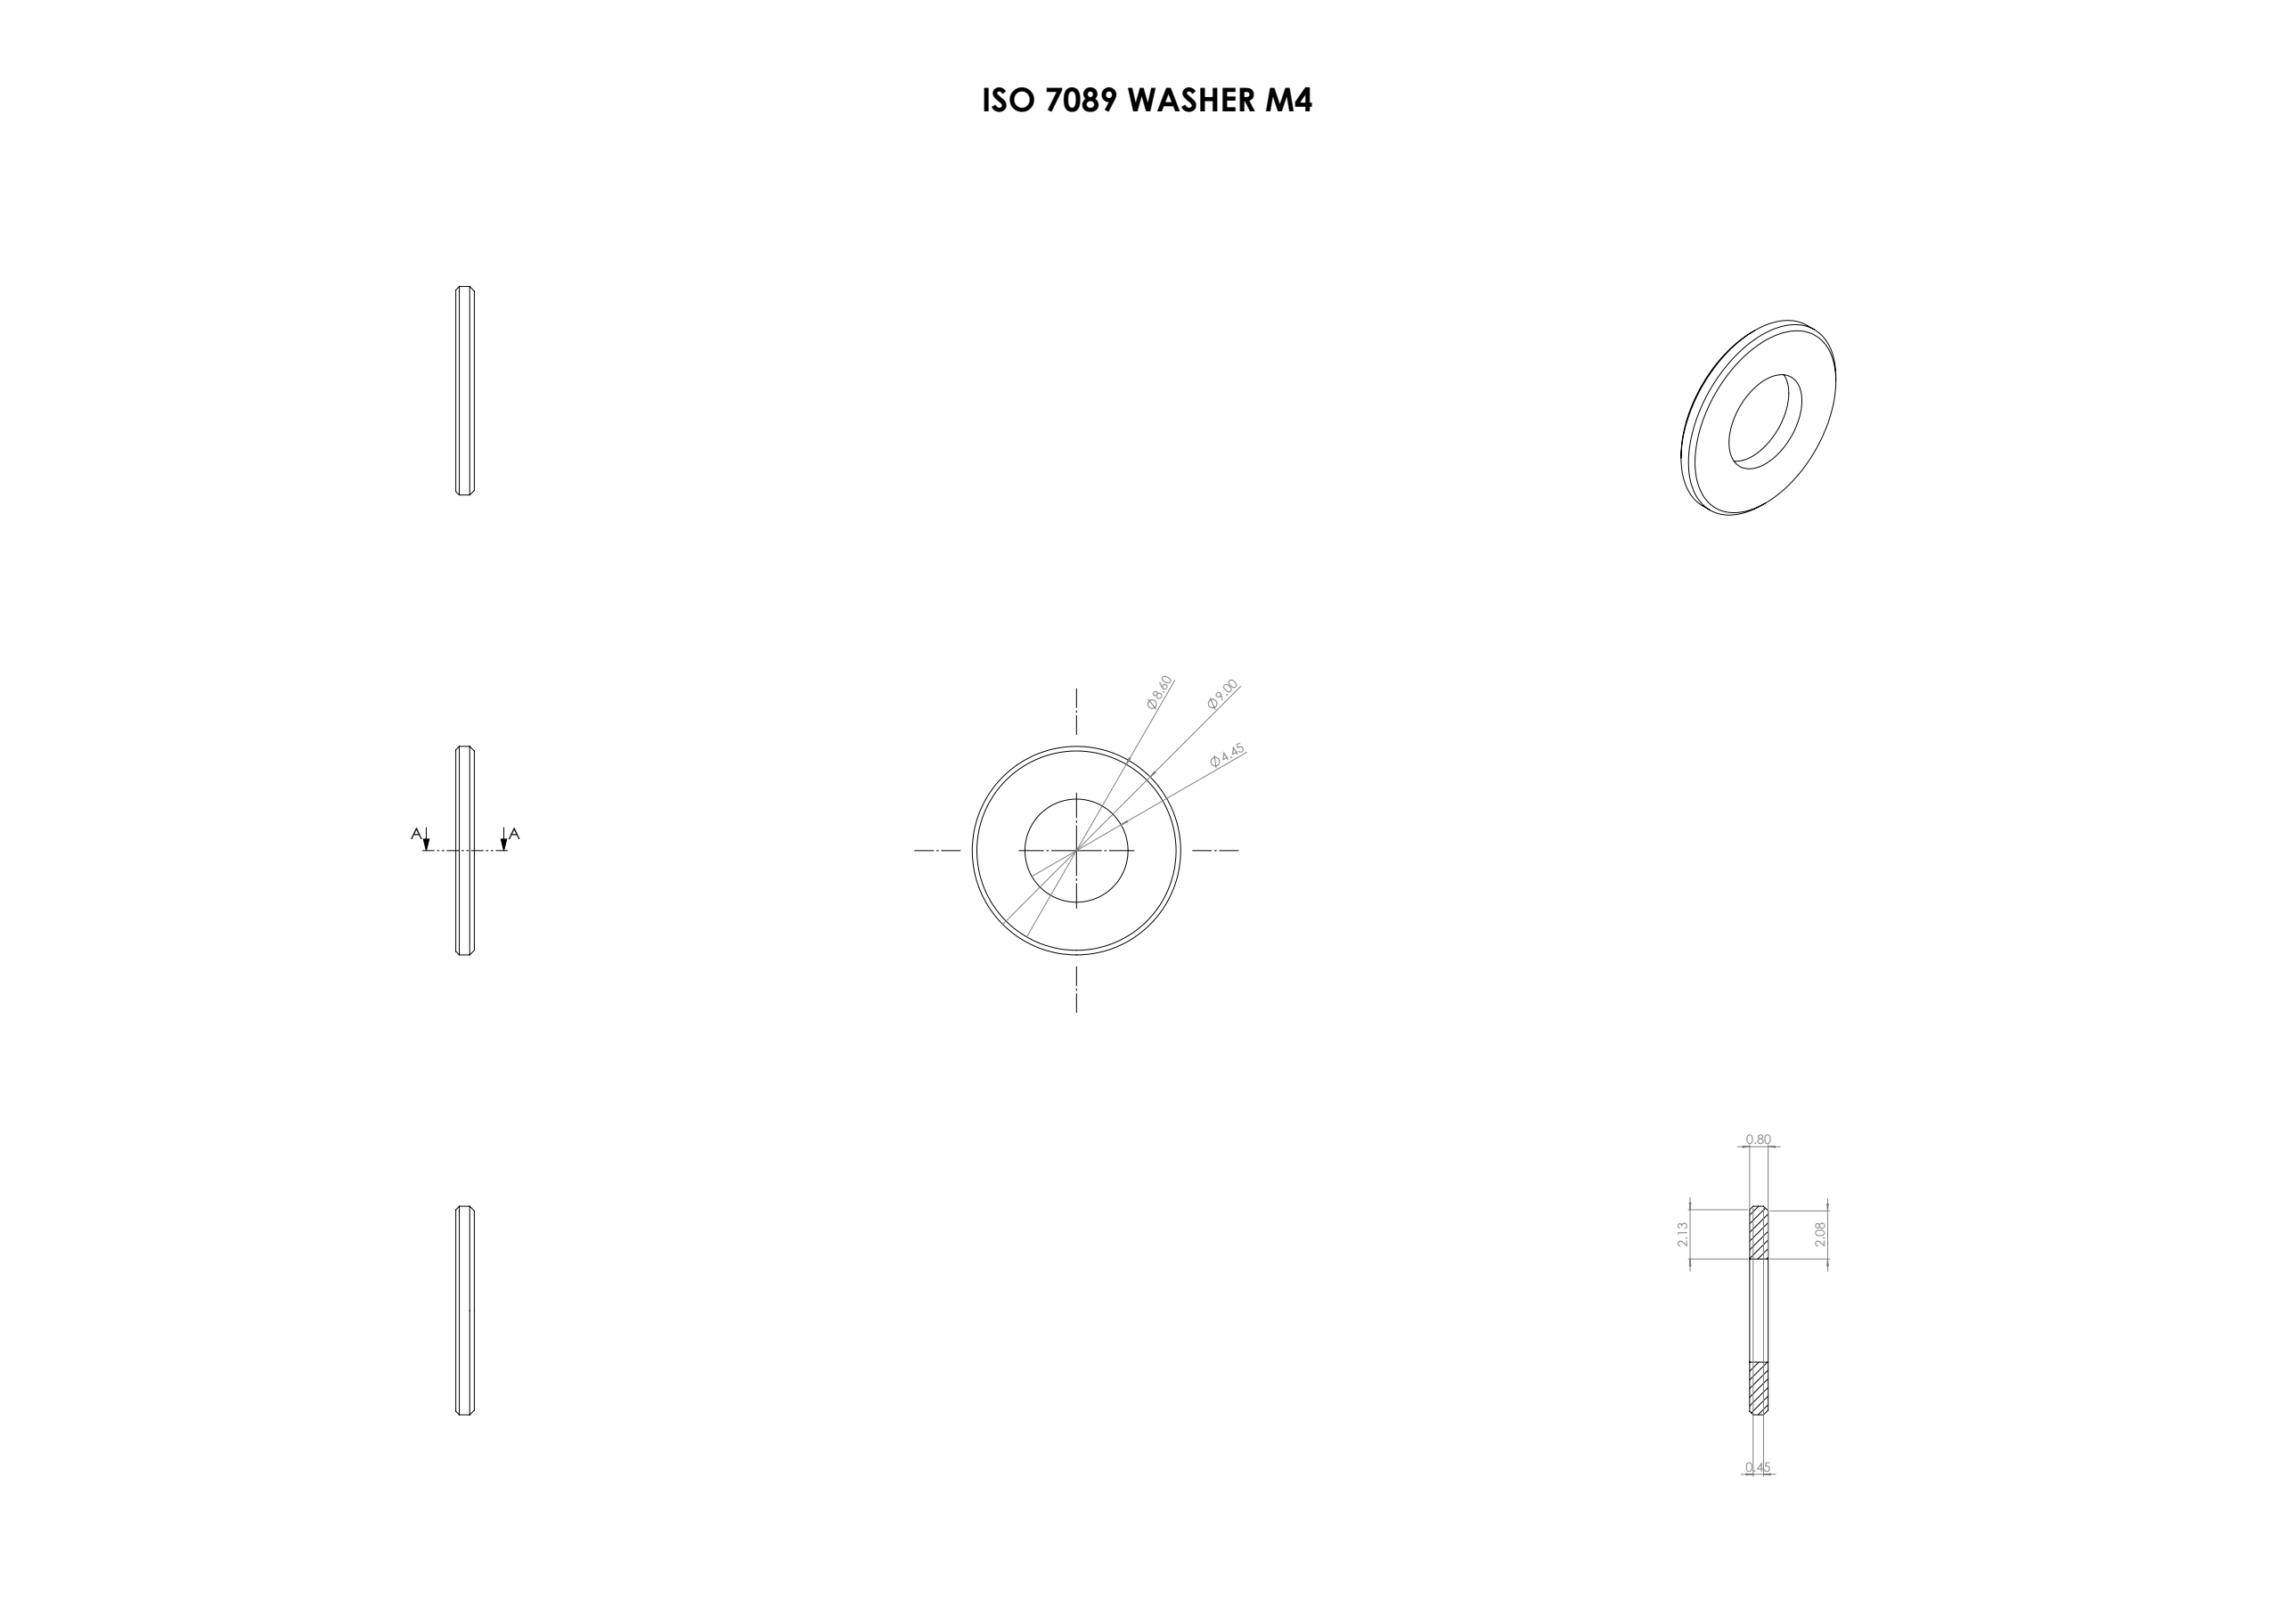
ISO-10303-21;
HEADER;
/* Generated by software containing ST-Developer
 * from STEP Tools, Inc. (www.steptools.com) 
 */

FILE_DESCRIPTION(
/* description */ (''),
/* implementation_level */ '2;1');

FILE_NAME(
/* name */ '15_ISO_7089_Washer_M4.step',
/* time_stamp */ '2026-10-21T01:56:51-07:00',
/* author */ (''),
/* organization */ (''),
/* preprocessor_version */ 'ST-DEVELOPER v20.2',
/* originating_system */ 'Autodesk Translation Framework v15.15.0.0',
/* authorisation */ '');

FILE_SCHEMA (('AUTOMOTIVE_DESIGN { 1 0 10303 214 3 1 1 }'));
ENDSEC;

DATA;
#10=MECHANICAL_DESIGN_GEOMETRIC_PRESENTATION_REPRESENTATION('',(#280),#82384);
#242=SHAPE_REPRESENTATION_RELATIONSHIP('SRR','None',#82476,#261);
#261=ADVANCED_BREP_SHAPE_REPRESENTATION('',(#299),#82375);
#280=STYLED_ITEM('',(#82638),#299);
#299=MANIFOLD_SOLID_BREP('Body1',#30671);
#576=CYLINDRICAL_SURFACE('',#32098,4.5);
#577=CYLINDRICAL_SURFACE('',#32102,2.225);
#1535=CIRCLE('',#32095,4.3);
#1536=CIRCLE('',#32096,4.5);
#1537=CIRCLE('',#32097,4.5);
#1538=CIRCLE('',#32099,4.5);
#1539=CIRCLE('',#32101,2.225);
#1540=CIRCLE('',#32103,2.225);
#1541=CIRCLE('',#32105,4.35);
#2037=CONICAL_SURFACE('',#32094,4.4,0.785398163397449);
#2038=CONICAL_SURFACE('',#32106,4.425,0.785398163397451);
#3486=FACE_BOUND('',#6345,.T.);
#3487=FACE_BOUND('',#6348,.T.);
#4384=FACE_OUTER_BOUND('',#6342,.T.);
#4385=FACE_OUTER_BOUND('',#6343,.T.);
#4386=FACE_OUTER_BOUND('',#6344,.T.);
#4387=FACE_OUTER_BOUND('',#6346,.T.);
#4388=FACE_OUTER_BOUND('',#6347,.T.);
#4389=FACE_OUTER_BOUND('',#6349,.T.);
#6342=EDGE_LOOP('',(#23061,#23062,#23063,#23064,#23065));
#6343=EDGE_LOOP('',(#23066,#23067,#23068,#23069,#23070));
#6344=EDGE_LOOP('',(#23071));
#6345=EDGE_LOOP('',(#23072));
#6346=EDGE_LOOP('',(#23073,#23074,#23075,#23076));
#6347=EDGE_LOOP('',(#23077));
#6348=EDGE_LOOP('',(#23078));
#6349=EDGE_LOOP('',(#23079,#23080,#23081,#23082));
#8479=LINE('',#49549,#10785);
#8480=LINE('',#49555,#10786);
#8481=LINE('',#49562,#10787);
#8482=LINE('',#49568,#10788);
#10785=VECTOR('',#36922,4.4);
#10786=VECTOR('',#36929,4.5);
#10787=VECTOR('',#36938,2.225);
#10788=VECTOR('',#36947,4.425);
#13187=VERTEX_POINT('',#49546);
#13188=VERTEX_POINT('',#49548);
#13189=VERTEX_POINT('',#49550);
#13190=VERTEX_POINT('',#49554);
#13191=VERTEX_POINT('',#49558);
#13192=VERTEX_POINT('',#49561);
#13193=VERTEX_POINT('',#49565);
#16752=EDGE_CURVE('',#13187,#13187,#1535,.T.);
#16753=EDGE_CURVE('',#13187,#13188,#8479,.T.);
#16754=EDGE_CURVE('',#13188,#13189,#1536,.T.);
#16755=EDGE_CURVE('',#13189,#13188,#1537,.T.);
#16756=EDGE_CURVE('',#13189,#13190,#8480,.T.);
#16757=EDGE_CURVE('',#13190,#13190,#1538,.T.);
#16758=EDGE_CURVE('',#13191,#13191,#1539,.T.);
#16759=EDGE_CURVE('',#13191,#13192,#8481,.T.);
#16760=EDGE_CURVE('',#13192,#13192,#1540,.T.);
#16761=EDGE_CURVE('',#13193,#13193,#1541,.T.);
#16762=EDGE_CURVE('',#13190,#13193,#8482,.T.);
#23061=ORIENTED_EDGE('',*,*,#16752,.T.);
#23062=ORIENTED_EDGE('',*,*,#16753,.T.);
#23063=ORIENTED_EDGE('',*,*,#16754,.T.);
#23064=ORIENTED_EDGE('',*,*,#16755,.T.);
#23065=ORIENTED_EDGE('',*,*,#16753,.F.);
#23066=ORIENTED_EDGE('',*,*,#16754,.F.);
#23067=ORIENTED_EDGE('',*,*,#16755,.F.);
#23068=ORIENTED_EDGE('',*,*,#16756,.T.);
#23069=ORIENTED_EDGE('',*,*,#16757,.T.);
#23070=ORIENTED_EDGE('',*,*,#16756,.F.);
#23071=ORIENTED_EDGE('',*,*,#16752,.F.);
#23072=ORIENTED_EDGE('',*,*,#16758,.F.);
#23073=ORIENTED_EDGE('',*,*,#16758,.T.);
#23074=ORIENTED_EDGE('',*,*,#16759,.T.);
#23075=ORIENTED_EDGE('',*,*,#16760,.F.);
#23076=ORIENTED_EDGE('',*,*,#16759,.F.);
#23077=ORIENTED_EDGE('',*,*,#16761,.F.);
#23078=ORIENTED_EDGE('',*,*,#16760,.T.);
#23079=ORIENTED_EDGE('',*,*,#16757,.F.);
#23080=ORIENTED_EDGE('',*,*,#16762,.T.);
#23081=ORIENTED_EDGE('',*,*,#16761,.T.);
#23082=ORIENTED_EDGE('',*,*,#16762,.F.);
#28476=PLANE('',#32100);
#28477=PLANE('',#32104);
#29712=ADVANCED_FACE('',(#4384),#2037,.T.);
#29713=ADVANCED_FACE('',(#4385),#576,.T.);
#29714=ADVANCED_FACE('',(#4386,#3486),#28476,.T.);
#29715=ADVANCED_FACE('',(#4387),#577,.F.);
#29716=ADVANCED_FACE('',(#4388,#3487),#28477,.T.);
#29717=ADVANCED_FACE('',(#4389),#2038,.T.);
#30671=CLOSED_SHELL('',(#29712,#29713,#29714,#29715,#29716,#29717));
#32093=AXIS2_PLACEMENT_3D('',#49544,#36916,#36917);
#32094=AXIS2_PLACEMENT_3D('',#49545,#36918,#36919);
#32095=AXIS2_PLACEMENT_3D('',#49547,#36920,#36921);
#32096=AXIS2_PLACEMENT_3D('',#49551,#36923,#36924);
#32097=AXIS2_PLACEMENT_3D('',#49552,#36925,#36926);
#32098=AXIS2_PLACEMENT_3D('',#49553,#36927,#36928);
#32099=AXIS2_PLACEMENT_3D('',#49556,#36930,#36931);
#32100=AXIS2_PLACEMENT_3D('',#49557,#36932,#36933);
#32101=AXIS2_PLACEMENT_3D('',#49559,#36934,#36935);
#32102=AXIS2_PLACEMENT_3D('',#49560,#36936,#36937);
#32103=AXIS2_PLACEMENT_3D('',#49563,#36939,#36940);
#32104=AXIS2_PLACEMENT_3D('',#49564,#36941,#36942);
#32105=AXIS2_PLACEMENT_3D('',#49566,#36943,#36944);
#32106=AXIS2_PLACEMENT_3D('',#49567,#36945,#36946);
#36916=DIRECTION('axis',(0.,0.,1.));
#36917=DIRECTION('refdir',(1.,0.,0.));
#36918=DIRECTION('center_axis',(-1.,0.,0.));
#36919=DIRECTION('ref_axis',(0.,-1.,0.));
#36920=DIRECTION('center_axis',(-1.,0.,0.));
#36921=DIRECTION('ref_axis',(0.,-1.,0.));
#36922=DIRECTION('',(-0.707106781186547,0.707106781186548,8.65956056235494E-17));
#36923=DIRECTION('center_axis',(1.,0.,0.));
#36924=DIRECTION('ref_axis',(0.,-1.,0.));
#36925=DIRECTION('center_axis',(1.,0.,0.));
#36926=DIRECTION('ref_axis',(0.,-1.,0.));
#36927=DIRECTION('center_axis',(1.,0.,0.));
#36928=DIRECTION('ref_axis',(0.,1.,0.));
#36929=DIRECTION('',(-1.,0.,0.));
#36930=DIRECTION('center_axis',(1.,0.,0.));
#36931=DIRECTION('ref_axis',(0.,0.,-1.));
#36932=DIRECTION('center_axis',(1.,0.,0.));
#36933=DIRECTION('ref_axis',(0.,0.,-1.));
#36934=DIRECTION('center_axis',(1.,0.,0.));
#36935=DIRECTION('ref_axis',(0.,0.,-1.));
#36936=DIRECTION('center_axis',(1.,0.,0.));
#36937=DIRECTION('ref_axis',(0.,1.,0.));
#36938=DIRECTION('',(-1.,0.,0.));
#36939=DIRECTION('center_axis',(1.,0.,0.));
#36940=DIRECTION('ref_axis',(0.,0.,-1.));
#36941=DIRECTION('center_axis',(-1.,0.,0.));
#36942=DIRECTION('ref_axis',(0.,0.,1.));
#36943=DIRECTION('center_axis',(1.,0.,0.));
#36944=DIRECTION('ref_axis',(0.,0.,-1.));
#36945=DIRECTION('center_axis',(1.,0.,0.));
#36946=DIRECTION('ref_axis',(0.,1.,0.));
#36947=DIRECTION('',(-0.707106781186546,0.707106781186549,8.65956056235496E-17));
#49544=CARTESIAN_POINT('',(0.,0.,0.));
#49545=CARTESIAN_POINT('Origin',(0.7,0.,0.));
#49546=CARTESIAN_POINT('',(0.8,4.3,-5.26598123633362E-16));
#49547=CARTESIAN_POINT('Origin',(0.8,0.,0.));
#49548=CARTESIAN_POINT('',(0.6,4.5,5.51091059616309E-16));
#49549=CARTESIAN_POINT('',(0.7,4.4,5.38844591624835E-16));
#49550=CARTESIAN_POINT('',(0.6,-4.5,-5.51091059616309E-16));
#49551=CARTESIAN_POINT('Origin',(0.6,0.,0.));
#49552=CARTESIAN_POINT('Origin',(0.6,0.,0.));
#49553=CARTESIAN_POINT('Origin',(0.475,0.,0.));
#49554=CARTESIAN_POINT('',(0.15,-4.5,-5.51091059616309E-16));
#49555=CARTESIAN_POINT('',(0.475,-4.5,-5.51091059616309E-16));
#49556=CARTESIAN_POINT('Origin',(0.15,0.,0.));
#49557=CARTESIAN_POINT('Origin',(0.8,2.225,0.));
#49558=CARTESIAN_POINT('',(0.8,-2.225,-2.72483912810286E-16));
#49559=CARTESIAN_POINT('Origin',(0.8,0.,0.));
#49560=CARTESIAN_POINT('Origin',(0.4,0.,0.));
#49561=CARTESIAN_POINT('',(0.,-2.225,-2.72483912810286E-16));
#49562=CARTESIAN_POINT('',(0.4,-2.225,-2.72483912810286E-16));
#49563=CARTESIAN_POINT('Origin',(0.,0.,0.));
#49564=CARTESIAN_POINT('Origin',(0.,4.35,0.));
#49565=CARTESIAN_POINT('',(-3.20923843055709E-16,-4.35,-5.32721357629099E-16));
#49566=CARTESIAN_POINT('Origin',(0.,0.,0.));
#49567=CARTESIAN_POINT('Origin',(0.0749999999999999,0.,0.));
#49568=CARTESIAN_POINT('',(0.0749999999999999,-4.425,-5.41906208622704E-16));
#82354=UNCERTAINTY_MEASURE_WITH_UNIT(LENGTH_MEASURE(0.01),#82385,
'DISTANCE_ACCURACY_VALUE',
'Maximum model space distance between geometric entities at asserted c
onnectivities');
#82363=UNCERTAINTY_MEASURE_WITH_UNIT(LENGTH_MEASURE(0.01),#82385,
'DISTANCE_ACCURACY_VALUE',
'Maximum model space distance between geometric entities at asserted c
onnectivities');
#82375=(
GEOMETRIC_REPRESENTATION_CONTEXT(3)
GLOBAL_UNCERTAINTY_ASSIGNED_CONTEXT((#82354))
GLOBAL_UNIT_ASSIGNED_CONTEXT((#82385,#82387,#82388))
REPRESENTATION_CONTEXT('','3D')
);
#82384=(
GEOMETRIC_REPRESENTATION_CONTEXT(3)
GLOBAL_UNCERTAINTY_ASSIGNED_CONTEXT((#82363))
GLOBAL_UNIT_ASSIGNED_CONTEXT((#82385,#82387,#82388))
REPRESENTATION_CONTEXT('','3D')
);
#82385=(
LENGTH_UNIT()
NAMED_UNIT(*)
SI_UNIT(.MILLI.,.METRE.)
);
#82387=(
NAMED_UNIT(*)
PLANE_ANGLE_UNIT()
SI_UNIT($,.RADIAN.)
);
#82388=(
NAMED_UNIT(*)
SI_UNIT($,.STERADIAN.)
SOLID_ANGLE_UNIT()
);
#82400=SHAPE_DEFINITION_REPRESENTATION(#82420,#82476);
#82420=PRODUCT_DEFINITION_SHAPE('',$,#82497);
#82476=SHAPE_REPRESENTATION('',(#32093),#82375);
#82485=PRODUCT_DEFINITION_CONTEXT('part definition',#82547,'design');
#82497=PRODUCT_DEFINITION('2026-10-20-12-38-28-563',
'15_ISO_7089_Washer_M4',#82517,#82485);
#82517=PRODUCT_DEFINITION_FORMATION('',$,#82560);
#82547=APPLICATION_CONTEXT(
'Core Data for Automotive Mechanical Design Process');
#82548=PRODUCT_CONTEXT('part definition',#82547,'mechanical');
#82560=PRODUCT('2026-10-20-12-38-28-563','15_ISO_7089_Washer_M4',$,(#82548));
#82632=COLOUR_RGB('Black',0.12,0.14,0.17);
#82633=FILL_AREA_STYLE_COLOUR('',#82632);
#82634=FILL_AREA_STYLE('',(#82633));
#82635=SURFACE_STYLE_FILL_AREA(#82634);
#82636=SURFACE_SIDE_STYLE('',(#82635));
#82637=SURFACE_STYLE_USAGE(.BOTH.,#82636);
#82638=PRESENTATION_STYLE_ASSIGNMENT((#82637));
ENDSEC;
END-ISO-10303-21;
